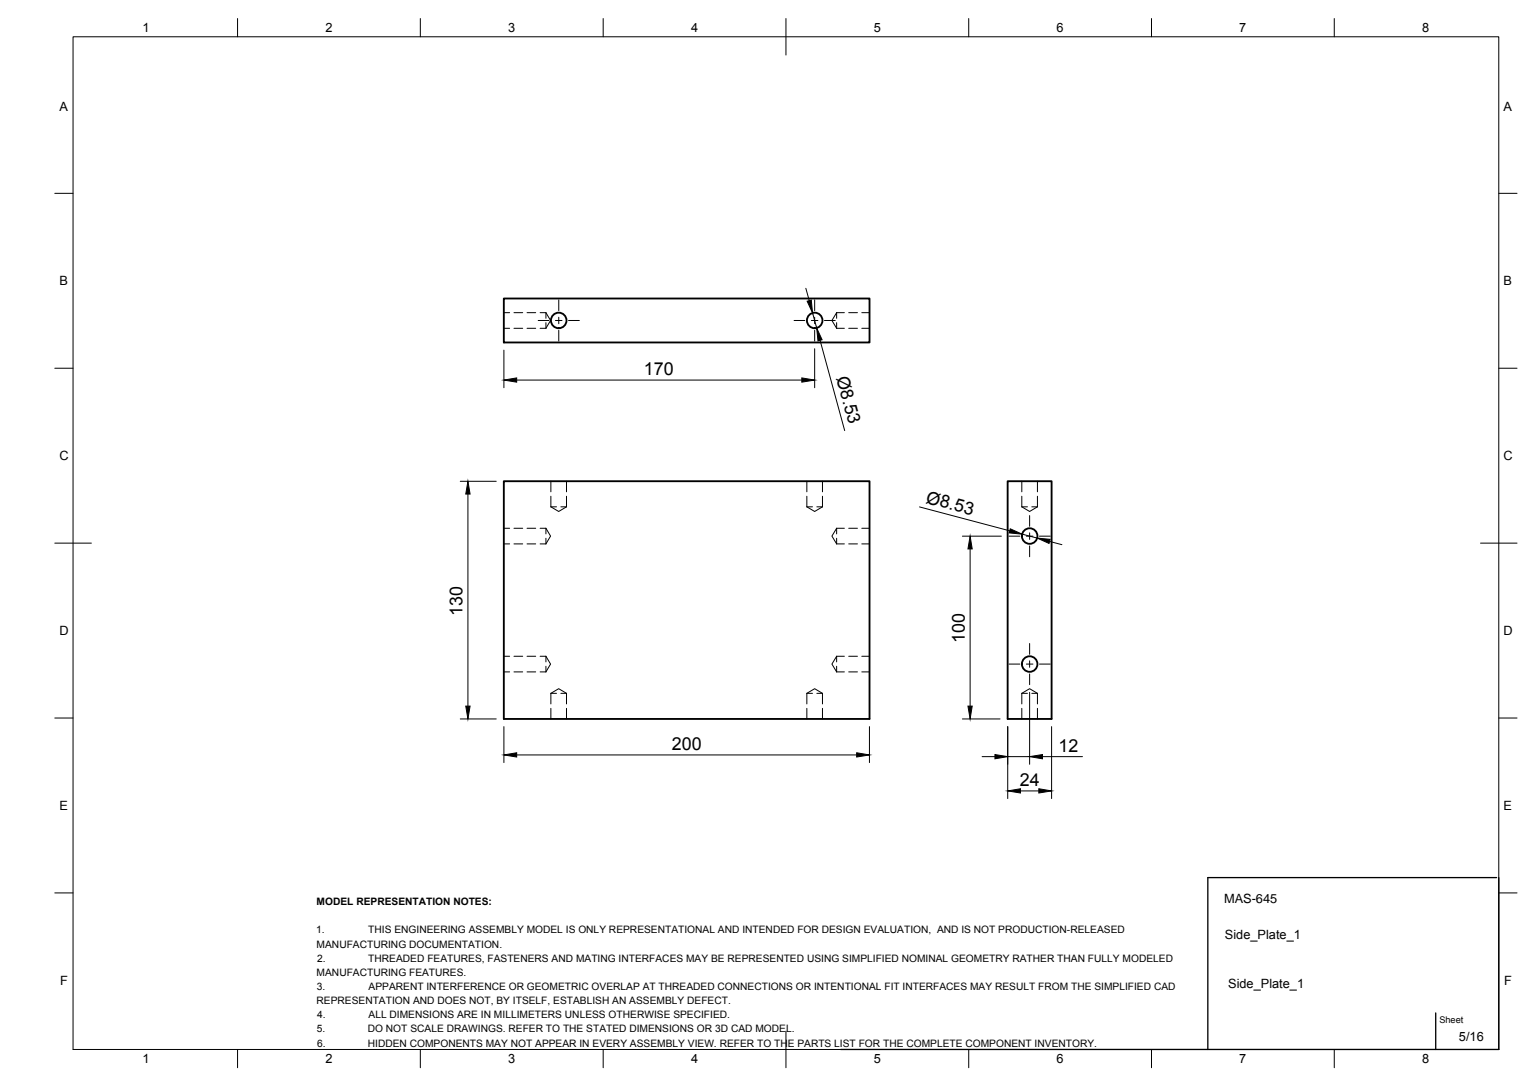
ISO-10303-21;
HEADER;
FILE_DESCRIPTION((''),'2;1');
FILE_NAME('Side_Plate_1.step','2026-10-09T10:54:55-07:00',(''),(''),'','','');
FILE_SCHEMA (('AUTOMOTIVE_DESIGN { 1 0 10303 214 3 1 1 }'));
ENDSEC;
DATA;
#10=MECHANICAL_DESIGN_GEOMETRIC_PRESENTATION_REPRESENTATION('',(#597),#63824);
#567=SHAPE_REPRESENTATION_RELATIONSHIP('SRR','None',#63881,#582) ;
#582=ADVANCED_BREP_SHAPE_REPRESENTATION('',(#612),#63811) ;
#597=STYLED_ITEM('',(#63963),#612) ;
#612=MANIFOLD_SOLID_BREP('Body1',#15496) ;
#687=FACE_BOUND('',#2566,.T.) ;
#688=FACE_BOUND('',#2567,.T.) ;
#689=FACE_BOUND('',#2574,.T.) ;
#690=FACE_BOUND('',#2575,.T.) ;
#691=FACE_BOUND('',#2578,.T.) ;
#692=FACE_BOUND('',#2579,.T.) ;
#693=FACE_BOUND('',#2581,.T.) ;
#694=FACE_BOUND('',#2582,.T.) ;
#860=PLANE('',#15878) ;
#861=PLANE('',#15887) ;
#862=PLANE('',#15888) ;
#863=PLANE('',#15889) ;
#864=PLANE('',#15890) ;
#865=PLANE('',#15891) ;
#1161=CYLINDRICAL_SURFACE('',#15856,4.263) ;
#1162=CYLINDRICAL_SURFACE('',#15860,4.263) ;
#1163=CYLINDRICAL_SURFACE('',#15864,4.263) ;
#1164=CYLINDRICAL_SURFACE('',#15868,4.263) ;
#1165=CYLINDRICAL_SURFACE('',#15872,4.263) ;
#1166=CYLINDRICAL_SURFACE('',#15876,4.263) ;
#1167=CYLINDRICAL_SURFACE('',#15881,4.263) ;
#1168=CYLINDRICAL_SURFACE('',#15885,4.263) ;
#1630=FACE_OUTER_BOUND('',#2553,.T.) ;
#1631=FACE_OUTER_BOUND('',#2554,.T.) ;
#1632=FACE_OUTER_BOUND('',#2555,.T.) ;
#1633=FACE_OUTER_BOUND('',#2556,.T.) ;
#1634=FACE_OUTER_BOUND('',#2557,.T.) ;
#1635=FACE_OUTER_BOUND('',#2558,.T.) ;
#1636=FACE_OUTER_BOUND('',#2559,.T.) ;
#1637=FACE_OUTER_BOUND('',#2560,.T.) ;
#1638=FACE_OUTER_BOUND('',#2561,.T.) ;
#1639=FACE_OUTER_BOUND('',#2562,.T.) ;
#1640=FACE_OUTER_BOUND('',#2563,.T.) ;
#1641=FACE_OUTER_BOUND('',#2564,.T.) ;
#1642=FACE_OUTER_BOUND('',#2565,.T.) ;
#1643=FACE_OUTER_BOUND('',#2568,.T.) ;
#1644=FACE_OUTER_BOUND('',#2569,.T.) ;
#1645=FACE_OUTER_BOUND('',#2570,.T.) ;
#1646=FACE_OUTER_BOUND('',#2571,.T.) ;
#1647=FACE_OUTER_BOUND('',#2572,.T.) ;
#1648=FACE_OUTER_BOUND('',#2573,.T.) ;
#1649=FACE_OUTER_BOUND('',#2576,.T.) ;
#1650=FACE_OUTER_BOUND('',#2577,.T.) ;
#1651=FACE_OUTER_BOUND('',#2580,.T.) ;
#2553=EDGE_LOOP('',(#10144,#10145,#10146)) ;
#2554=EDGE_LOOP('',(#10147,#10148,#10149,#10150)) ;
#2555=EDGE_LOOP('',(#10151,#10152,#10153)) ;
#2556=EDGE_LOOP('',(#10154,#10155,#10156,#10157)) ;
#2557=EDGE_LOOP('',(#10158,#10159,#10160)) ;
#2558=EDGE_LOOP('',(#10161,#10162,#10163,#10164)) ;
#2559=EDGE_LOOP('',(#10165,#10166,#10167)) ;
#2560=EDGE_LOOP('',(#10168,#10169,#10170,#10171)) ;
#2561=EDGE_LOOP('',(#10172,#10173,#10174)) ;
#2562=EDGE_LOOP('',(#10175,#10176,#10177,#10178)) ;
#2563=EDGE_LOOP('',(#10179,#10180,#10181)) ;
#2564=EDGE_LOOP('',(#10182,#10183,#10184,#10185)) ;
#2565=EDGE_LOOP('',(#10186,#10187,#10188,#10189)) ;
#2566=EDGE_LOOP('',(#10190)) ;
#2567=EDGE_LOOP('',(#10191)) ;
#2568=EDGE_LOOP('',(#10192,#10193,#10194)) ;
#2569=EDGE_LOOP('',(#10195,#10196,#10197,#10198)) ;
#2570=EDGE_LOOP('',(#10199,#10200,#10201)) ;
#2571=EDGE_LOOP('',(#10202,#10203,#10204,#10205)) ;
#2572=EDGE_LOOP('',(#10206,#10207,#10208,#10209)) ;
#2573=EDGE_LOOP('',(#10210,#10211,#10212,#10213)) ;
#2574=EDGE_LOOP('',(#10214)) ;
#2575=EDGE_LOOP('',(#10215)) ;
#2576=EDGE_LOOP('',(#10216,#10217,#10218,#10219)) ;
#2577=EDGE_LOOP('',(#10220,#10221,#10222,#10223)) ;
#2578=EDGE_LOOP('',(#10224)) ;
#2579=EDGE_LOOP('',(#10225)) ;
#2580=EDGE_LOOP('',(#10226,#10227,#10228,#10229)) ;
#2581=EDGE_LOOP('',(#10230)) ;
#2582=EDGE_LOOP('',(#10231)) ;
#3564=CIRCLE('',#15855,4.263) ;
#3565=CIRCLE('',#15857,4.263) ;
#3566=CIRCLE('',#15859,4.263) ;
#3567=CIRCLE('',#15861,4.263) ;
#3568=CIRCLE('',#15863,4.263) ;
#3569=CIRCLE('',#15865,4.263) ;
#3570=CIRCLE('',#15867,4.263) ;
#3571=CIRCLE('',#15869,4.263) ;
#3572=CIRCLE('',#15871,4.263) ;
#3573=CIRCLE('',#15873,4.263) ;
#3574=CIRCLE('',#15875,4.263) ;
#3575=CIRCLE('',#15877,4.263) ;
#3576=CIRCLE('',#15880,4.263) ;
#3577=CIRCLE('',#15882,4.263) ;
#3578=CIRCLE('',#15884,4.263) ;
#3579=CIRCLE('',#15886,4.263) ;
#4771=LINE('',#23393,#5427) ;
#4772=LINE('',#23398,#5428) ;
#4773=LINE('',#23402,#5429) ;
#4774=LINE('',#23407,#5430) ;
#4775=LINE('',#23411,#5431) ;
#4776=LINE('',#23416,#5432) ;
#4777=LINE('',#23420,#5433) ;
#4778=LINE('',#23425,#5434) ;
#4779=LINE('',#23429,#5435) ;
#4780=LINE('',#23433,#5436) ;
#4781=LINE('',#23438,#5437) ;
#4782=LINE('',#23442,#5438) ;
#4783=LINE('',#23447,#5439) ;
#4784=LINE('',#23449,#5440) ;
#4785=LINE('',#23451,#5441) ;
#4786=LINE('',#23452,#5442) ;
#4787=LINE('',#23456,#5443) ;
#4788=LINE('',#23461,#5444) ;
#4789=LINE('',#23465,#5445) ;
#4790=LINE('',#23470,#5446) ;
#4791=LINE('',#23474,#5447) ;
#4792=LINE('',#23475,#5448) ;
#4793=LINE('',#23476,#5449) ;
#4794=LINE('',#23479,#5450) ;
#4795=LINE('',#23480,#5451) ;
#4796=LINE('',#23483,#5452) ;
#4797=LINE('',#23484,#5453) ;
#4798=LINE('',#23486,#5454) ;
#5427=VECTOR('',#18343,2.42186816158307) ;
#5428=VECTOR('',#18350,4.263) ;
#5429=VECTOR('',#18353,2.42186816158307) ;
#5430=VECTOR('',#18360,4.263) ;
#5431=VECTOR('',#18363,2.42186816158307) ;
#5432=VECTOR('',#18370,4.263) ;
#5433=VECTOR('',#18373,2.42186816158307) ;
#5434=VECTOR('',#18380,4.263) ;
#5435=VECTOR('',#18383,2.42186816158307) ;
#5436=VECTOR('',#18388,4.263) ;
#5437=VECTOR('',#18393,2.42186816158307) ;
#5438=VECTOR('',#18398,4.263) ;
#5439=VECTOR('',#18403,10.) ;
#5440=VECTOR('',#18404,10.) ;
#5441=VECTOR('',#18405,10.) ;
#5442=VECTOR('',#18406,10.) ;
#5443=VECTOR('',#18409,2.42186816158307) ;
#5444=VECTOR('',#18416,4.263) ;
#5445=VECTOR('',#18419,2.42186816158307) ;
#5446=VECTOR('',#18426,4.263) ;
#5447=VECTOR('',#18429,10.) ;
#5448=VECTOR('',#18430,10.) ;
#5449=VECTOR('',#18431,10.) ;
#5450=VECTOR('',#18434,10.) ;
#5451=VECTOR('',#18435,10.) ;
#5452=VECTOR('',#18438,10.) ;
#5453=VECTOR('',#18439,10.) ;
#5454=VECTOR('',#18442,10.) ;
#6120=VERTEX_POINT('',#23391) ;
#6121=VERTEX_POINT('',#23392) ;
#6122=VERTEX_POINT('',#23396) ;
#6123=VERTEX_POINT('',#23400) ;
#6124=VERTEX_POINT('',#23401) ;
#6125=VERTEX_POINT('',#23405) ;
#6126=VERTEX_POINT('',#23409) ;
#6127=VERTEX_POINT('',#23410) ;
#6128=VERTEX_POINT('',#23414) ;
#6129=VERTEX_POINT('',#23418) ;
#6130=VERTEX_POINT('',#23419) ;
#6131=VERTEX_POINT('',#23423) ;
#6132=VERTEX_POINT('',#23427) ;
#6133=VERTEX_POINT('',#23428) ;
#6134=VERTEX_POINT('',#23432) ;
#6135=VERTEX_POINT('',#23436) ;
#6136=VERTEX_POINT('',#23437) ;
#6137=VERTEX_POINT('',#23441) ;
#6138=VERTEX_POINT('',#23445) ;
#6139=VERTEX_POINT('',#23446) ;
#6140=VERTEX_POINT('',#23448) ;
#6141=VERTEX_POINT('',#23450) ;
#6142=VERTEX_POINT('',#23454) ;
#6143=VERTEX_POINT('',#23455) ;
#6144=VERTEX_POINT('',#23459) ;
#6145=VERTEX_POINT('',#23463) ;
#6146=VERTEX_POINT('',#23464) ;
#6147=VERTEX_POINT('',#23468) ;
#6148=VERTEX_POINT('',#23472) ;
#6149=VERTEX_POINT('',#23473) ;
#6150=VERTEX_POINT('',#23478) ;
#6151=VERTEX_POINT('',#23482) ;
#7626=EDGE_CURVE('',#6120,#6121,#4771,.T.) ;
#7627=EDGE_CURVE('',#6121,#6121,#3564,.T.) ;
#7628=EDGE_CURVE('',#6122,#6122,#3565,.T.) ;
#7629=EDGE_CURVE('',#6122,#6121,#4772,.T.) ;
#7630=EDGE_CURVE('',#6123,#6124,#4773,.T.) ;
#7631=EDGE_CURVE('',#6124,#6124,#3566,.T.) ;
#7632=EDGE_CURVE('',#6125,#6125,#3567,.T.) ;
#7633=EDGE_CURVE('',#6125,#6124,#4774,.T.) ;
#7634=EDGE_CURVE('',#6126,#6127,#4775,.T.) ;
#7635=EDGE_CURVE('',#6127,#6127,#3568,.T.) ;
#7636=EDGE_CURVE('',#6128,#6128,#3569,.T.) ;
#7637=EDGE_CURVE('',#6128,#6127,#4776,.T.) ;
#7638=EDGE_CURVE('',#6129,#6130,#4777,.T.) ;
#7639=EDGE_CURVE('',#6130,#6130,#3570,.T.) ;
#7640=EDGE_CURVE('',#6131,#6131,#3571,.T.) ;
#7641=EDGE_CURVE('',#6131,#6130,#4778,.T.) ;
#7642=EDGE_CURVE('',#6132,#6133,#4779,.T.) ;
#7643=EDGE_CURVE('',#6133,#6133,#3572,.T.) ;
#7644=EDGE_CURVE('',#6133,#6134,#4780,.T.) ;
#7645=EDGE_CURVE('',#6134,#6134,#3573,.F.) ;
#7646=EDGE_CURVE('',#6135,#6136,#4781,.T.) ;
#7647=EDGE_CURVE('',#6136,#6136,#3574,.T.) ;
#7648=EDGE_CURVE('',#6136,#6137,#4782,.T.) ;
#7649=EDGE_CURVE('',#6137,#6137,#3575,.F.) ;
#7650=EDGE_CURVE('',#6138,#6139,#4783,.T.) ;
#7651=EDGE_CURVE('',#6140,#6138,#4784,.T.) ;
#7652=EDGE_CURVE('',#6141,#6140,#4785,.T.) ;
#7653=EDGE_CURVE('',#6139,#6141,#4786,.T.) ;
#7654=EDGE_CURVE('',#6142,#6143,#4787,.T.) ;
#7655=EDGE_CURVE('',#6143,#6143,#3576,.T.) ;
#7656=EDGE_CURVE('',#6144,#6144,#3577,.F.) ;
#7657=EDGE_CURVE('',#6144,#6143,#4788,.T.) ;
#7658=EDGE_CURVE('',#6145,#6146,#4789,.T.) ;
#7659=EDGE_CURVE('',#6146,#6146,#3578,.T.) ;
#7660=EDGE_CURVE('',#6147,#6147,#3579,.F.) ;
#7661=EDGE_CURVE('',#6147,#6146,#4790,.T.) ;
#7662=EDGE_CURVE('',#6148,#6149,#4791,.T.) ;
#7663=EDGE_CURVE('',#6148,#6139,#4792,.T.) ;
#7664=EDGE_CURVE('',#6149,#6141,#4793,.T.) ;
#7665=EDGE_CURVE('',#6149,#6150,#4794,.T.) ;
#7666=EDGE_CURVE('',#6150,#6140,#4795,.T.) ;
#7667=EDGE_CURVE('',#6150,#6151,#4796,.T.) ;
#7668=EDGE_CURVE('',#6151,#6138,#4797,.T.) ;
#7669=EDGE_CURVE('',#6151,#6148,#4798,.T.) ;
#10144=ORIENTED_EDGE('',*,*,#7626,.T.) ;
#10145=ORIENTED_EDGE('',*,*,#7627,.F.) ;
#10146=ORIENTED_EDGE('',*,*,#7626,.F.) ;
#10147=ORIENTED_EDGE('',*,*,#7628,.F.) ;
#10148=ORIENTED_EDGE('',*,*,#7629,.T.) ;
#10149=ORIENTED_EDGE('',*,*,#7627,.T.) ;
#10150=ORIENTED_EDGE('',*,*,#7629,.F.) ;
#10151=ORIENTED_EDGE('',*,*,#7630,.T.) ;
#10152=ORIENTED_EDGE('',*,*,#7631,.F.) ;
#10153=ORIENTED_EDGE('',*,*,#7630,.F.) ;
#10154=ORIENTED_EDGE('',*,*,#7632,.F.) ;
#10155=ORIENTED_EDGE('',*,*,#7633,.T.) ;
#10156=ORIENTED_EDGE('',*,*,#7631,.T.) ;
#10157=ORIENTED_EDGE('',*,*,#7633,.F.) ;
#10158=ORIENTED_EDGE('',*,*,#7634,.T.) ;
#10159=ORIENTED_EDGE('',*,*,#7635,.F.) ;
#10160=ORIENTED_EDGE('',*,*,#7634,.F.) ;
#10161=ORIENTED_EDGE('',*,*,#7636,.F.) ;
#10162=ORIENTED_EDGE('',*,*,#7637,.T.) ;
#10163=ORIENTED_EDGE('',*,*,#7635,.T.) ;
#10164=ORIENTED_EDGE('',*,*,#7637,.F.) ;
#10165=ORIENTED_EDGE('',*,*,#7638,.T.) ;
#10166=ORIENTED_EDGE('',*,*,#7639,.F.) ;
#10167=ORIENTED_EDGE('',*,*,#7638,.F.) ;
#10168=ORIENTED_EDGE('',*,*,#7640,.F.) ;
#10169=ORIENTED_EDGE('',*,*,#7641,.T.) ;
#10170=ORIENTED_EDGE('',*,*,#7639,.T.) ;
#10171=ORIENTED_EDGE('',*,*,#7641,.F.) ;
#10172=ORIENTED_EDGE('',*,*,#7642,.T.) ;
#10173=ORIENTED_EDGE('',*,*,#7643,.T.) ;
#10174=ORIENTED_EDGE('',*,*,#7642,.F.) ;
#10175=ORIENTED_EDGE('',*,*,#7643,.F.) ;
#10176=ORIENTED_EDGE('',*,*,#7644,.T.) ;
#10177=ORIENTED_EDGE('',*,*,#7645,.T.) ;
#10178=ORIENTED_EDGE('',*,*,#7644,.F.) ;
#10179=ORIENTED_EDGE('',*,*,#7646,.T.) ;
#10180=ORIENTED_EDGE('',*,*,#7647,.T.) ;
#10181=ORIENTED_EDGE('',*,*,#7646,.F.) ;
#10182=ORIENTED_EDGE('',*,*,#7647,.F.) ;
#10183=ORIENTED_EDGE('',*,*,#7648,.T.) ;
#10184=ORIENTED_EDGE('',*,*,#7649,.T.) ;
#10185=ORIENTED_EDGE('',*,*,#7648,.F.) ;
#10186=ORIENTED_EDGE('',*,*,#7650,.F.) ;
#10187=ORIENTED_EDGE('',*,*,#7651,.F.) ;
#10188=ORIENTED_EDGE('',*,*,#7652,.F.) ;
#10189=ORIENTED_EDGE('',*,*,#7653,.F.) ;
#10190=ORIENTED_EDGE('',*,*,#7645,.F.) ;
#10191=ORIENTED_EDGE('',*,*,#7649,.F.) ;
#10192=ORIENTED_EDGE('',*,*,#7654,.T.) ;
#10193=ORIENTED_EDGE('',*,*,#7655,.F.) ;
#10194=ORIENTED_EDGE('',*,*,#7654,.F.) ;
#10195=ORIENTED_EDGE('',*,*,#7656,.F.) ;
#10196=ORIENTED_EDGE('',*,*,#7657,.T.) ;
#10197=ORIENTED_EDGE('',*,*,#7655,.T.) ;
#10198=ORIENTED_EDGE('',*,*,#7657,.F.) ;
#10199=ORIENTED_EDGE('',*,*,#7658,.T.) ;
#10200=ORIENTED_EDGE('',*,*,#7659,.F.) ;
#10201=ORIENTED_EDGE('',*,*,#7658,.F.) ;
#10202=ORIENTED_EDGE('',*,*,#7660,.F.) ;
#10203=ORIENTED_EDGE('',*,*,#7661,.T.) ;
#10204=ORIENTED_EDGE('',*,*,#7659,.T.) ;
#10205=ORIENTED_EDGE('',*,*,#7661,.F.) ;
#10206=ORIENTED_EDGE('',*,*,#7662,.F.) ;
#10207=ORIENTED_EDGE('',*,*,#7663,.T.) ;
#10208=ORIENTED_EDGE('',*,*,#7653,.T.) ;
#10209=ORIENTED_EDGE('',*,*,#7664,.F.) ;
#10210=ORIENTED_EDGE('',*,*,#7665,.F.) ;
#10211=ORIENTED_EDGE('',*,*,#7664,.T.) ;
#10212=ORIENTED_EDGE('',*,*,#7652,.T.) ;
#10213=ORIENTED_EDGE('',*,*,#7666,.F.) ;
#10214=ORIENTED_EDGE('',*,*,#7628,.T.) ;
#10215=ORIENTED_EDGE('',*,*,#7632,.T.) ;
#10216=ORIENTED_EDGE('',*,*,#7667,.F.) ;
#10217=ORIENTED_EDGE('',*,*,#7666,.T.) ;
#10218=ORIENTED_EDGE('',*,*,#7651,.T.) ;
#10219=ORIENTED_EDGE('',*,*,#7668,.F.) ;
#10220=ORIENTED_EDGE('',*,*,#7669,.F.) ;
#10221=ORIENTED_EDGE('',*,*,#7668,.T.) ;
#10222=ORIENTED_EDGE('',*,*,#7650,.T.) ;
#10223=ORIENTED_EDGE('',*,*,#7663,.F.) ;
#10224=ORIENTED_EDGE('',*,*,#7636,.T.) ;
#10225=ORIENTED_EDGE('',*,*,#7640,.T.) ;
#10226=ORIENTED_EDGE('',*,*,#7669,.T.) ;
#10227=ORIENTED_EDGE('',*,*,#7662,.T.) ;
#10228=ORIENTED_EDGE('',*,*,#7665,.T.) ;
#10229=ORIENTED_EDGE('',*,*,#7667,.T.) ;
#10230=ORIENTED_EDGE('',*,*,#7656,.T.) ;
#10231=ORIENTED_EDGE('',*,*,#7660,.T.) ;
#14508=CONICAL_SURFACE('',#15854,2.42186816158307,1.02974425867665) ;
#14509=CONICAL_SURFACE('',#15858,2.42186816158307,1.02974425867665) ;
#14510=CONICAL_SURFACE('',#15862,2.42186816158307,1.02974425867665) ;
#14511=CONICAL_SURFACE('',#15866,2.42186816158307,1.02974425867665) ;
#14512=CONICAL_SURFACE('',#15870,2.42186816158307,1.02974425867665) ;
#14513=CONICAL_SURFACE('',#15874,2.42186816158307,1.02974425867665) ;
#14514=CONICAL_SURFACE('',#15879,2.42186816158307,1.02974425867665) ;
#14515=CONICAL_SURFACE('',#15883,2.42186816158307,1.02974425867665) ;
#14718=ADVANCED_FACE('',(#1630),#14508,.F.) ;
#14719=ADVANCED_FACE('',(#1631),#1161,.F.) ;
#14720=ADVANCED_FACE('',(#1632),#14509,.F.) ;
#14721=ADVANCED_FACE('',(#1633),#1162,.F.) ;
#14722=ADVANCED_FACE('',(#1634),#14510,.F.) ;
#14723=ADVANCED_FACE('',(#1635),#1163,.F.) ;
#14724=ADVANCED_FACE('',(#1636),#14511,.F.) ;
#14725=ADVANCED_FACE('',(#1637),#1164,.F.) ;
#14726=ADVANCED_FACE('',(#1638),#14512,.F.) ;
#14727=ADVANCED_FACE('',(#1639),#1165,.F.) ;
#14728=ADVANCED_FACE('',(#1640),#14513,.F.) ;
#14729=ADVANCED_FACE('',(#1641),#1166,.F.) ;
#14730=ADVANCED_FACE('',(#1642,#687,#688),#860,.T.) ;
#14731=ADVANCED_FACE('',(#1643),#14514,.F.) ;
#14732=ADVANCED_FACE('',(#1644),#1167,.F.) ;
#14733=ADVANCED_FACE('',(#1645),#14515,.F.) ;
#14734=ADVANCED_FACE('',(#1646),#1168,.F.) ;
#14735=ADVANCED_FACE('',(#1647),#861,.T.) ;
#14736=ADVANCED_FACE('',(#1648,#689,#690),#862,.T.) ;
#14737=ADVANCED_FACE('',(#1649),#863,.T.) ;
#14738=ADVANCED_FACE('',(#1650,#691,#692),#864,.T.) ;
#14739=ADVANCED_FACE('',(#1651,#693,#694),#865,.F.) ;
#15496=CLOSED_SHELL('',(#14718,#14719,#14720,#14721,#14722,#14723,#14724,
#14725,#14726,#14727,#14728,#14729,#14730,#14731,#14732,#14733,#14734,#14735,
#14736,#14737,#14738,#14739)) ;
#15853=AXIS2_PLACEMENT_3D('',#23389,#18339,#18340) ;
#15854=AXIS2_PLACEMENT_3D('',#23390,#18341,#18342) ;
#15855=AXIS2_PLACEMENT_3D('',#23394,#18344,#18345) ;
#15856=AXIS2_PLACEMENT_3D('',#23395,#18346,#18347) ;
#15857=AXIS2_PLACEMENT_3D('',#23397,#18348,#18349) ;
#15858=AXIS2_PLACEMENT_3D('',#23399,#18351,#18352) ;
#15859=AXIS2_PLACEMENT_3D('',#23403,#18354,#18355) ;
#15860=AXIS2_PLACEMENT_3D('',#23404,#18356,#18357) ;
#15861=AXIS2_PLACEMENT_3D('',#23406,#18358,#18359) ;
#15862=AXIS2_PLACEMENT_3D('',#23408,#18361,#18362) ;
#15863=AXIS2_PLACEMENT_3D('',#23412,#18364,#18365) ;
#15864=AXIS2_PLACEMENT_3D('',#23413,#18366,#18367) ;
#15865=AXIS2_PLACEMENT_3D('',#23415,#18368,#18369) ;
#15866=AXIS2_PLACEMENT_3D('',#23417,#18371,#18372) ;
#15867=AXIS2_PLACEMENT_3D('',#23421,#18374,#18375) ;
#15868=AXIS2_PLACEMENT_3D('',#23422,#18376,#18377) ;
#15869=AXIS2_PLACEMENT_3D('',#23424,#18378,#18379) ;
#15870=AXIS2_PLACEMENT_3D('',#23426,#18381,#18382) ;
#15871=AXIS2_PLACEMENT_3D('',#23430,#18384,#18385) ;
#15872=AXIS2_PLACEMENT_3D('',#23431,#18386,#18387) ;
#15873=AXIS2_PLACEMENT_3D('',#23434,#18389,#18390) ;
#15874=AXIS2_PLACEMENT_3D('',#23435,#18391,#18392) ;
#15875=AXIS2_PLACEMENT_3D('',#23439,#18394,#18395) ;
#15876=AXIS2_PLACEMENT_3D('',#23440,#18396,#18397) ;
#15877=AXIS2_PLACEMENT_3D('',#23443,#18399,#18400) ;
#15878=AXIS2_PLACEMENT_3D('',#23444,#18401,#18402) ;
#15879=AXIS2_PLACEMENT_3D('',#23453,#18407,#18408) ;
#15880=AXIS2_PLACEMENT_3D('',#23457,#18410,#18411) ;
#15881=AXIS2_PLACEMENT_3D('',#23458,#18412,#18413) ;
#15882=AXIS2_PLACEMENT_3D('',#23460,#18414,#18415) ;
#15883=AXIS2_PLACEMENT_3D('',#23462,#18417,#18418) ;
#15884=AXIS2_PLACEMENT_3D('',#23466,#18420,#18421) ;
#15885=AXIS2_PLACEMENT_3D('',#23467,#18422,#18423) ;
#15886=AXIS2_PLACEMENT_3D('',#23469,#18424,#18425) ;
#15887=AXIS2_PLACEMENT_3D('',#23471,#18427,#18428) ;
#15888=AXIS2_PLACEMENT_3D('',#23477,#18432,#18433) ;
#15889=AXIS2_PLACEMENT_3D('',#23481,#18436,#18437) ;
#15890=AXIS2_PLACEMENT_3D('',#23485,#18440,#18441) ;
#15891=AXIS2_PLACEMENT_3D('',#23487,#18443,#18444) ;
#18339=DIRECTION('axis',(0.,0.,1.)) ;
#18340=DIRECTION('refdir',(1.,0.,0.)) ;
#18341=DIRECTION('center_axis',(-9.473903143468E-16,1.,0.)) ;
#18342=DIRECTION('ref_axis',(0.,0.,1.)) ;
#18343=DIRECTION('',(-5.92914802803472E-16,0.515038074910058,-0.85716730070211)) ;
#18344=DIRECTION('center_axis',(9.473903143468E-16,-1.,0.)) ;
#18345=DIRECTION('ref_axis',(0.,0.,1.)) ;
#18346=DIRECTION('center_axis',(9.473903143468E-16,-1.,0.)) ;
#18347=DIRECTION('ref_axis',(0.,0.,1.)) ;
#18348=DIRECTION('center_axis',(9.47390314346801E-16,-1.,0.)) ;
#18349=DIRECTION('ref_axis',(0.,0.,1.)) ;
#18350=DIRECTION('',(9.473903143468E-16,-1.,0.)) ;
#18351=DIRECTION('center_axis',(-9.473903143468E-16,1.,0.)) ;
#18352=DIRECTION('ref_axis',(0.,0.,1.)) ;
#18353=DIRECTION('',(-5.92914802803472E-16,0.515038074910058,-0.85716730070211)) ;
#18354=DIRECTION('center_axis',(9.473903143468E-16,-1.,0.)) ;
#18355=DIRECTION('ref_axis',(0.,0.,1.)) ;
#18356=DIRECTION('center_axis',(9.473903143468E-16,-1.,0.)) ;
#18357=DIRECTION('ref_axis',(0.,0.,1.)) ;
#18358=DIRECTION('center_axis',(9.47390314346801E-16,-1.,0.)) ;
#18359=DIRECTION('ref_axis',(0.,0.,1.)) ;
#18360=DIRECTION('',(9.473903143468E-16,-1.,0.)) ;
#18361=DIRECTION('center_axis',(-3.5527136788005E-16,-1.,0.)) ;
#18362=DIRECTION('ref_axis',(0.,0.,-1.)) ;
#18363=DIRECTION('',(-2.87951000497466E-16,-0.515038074910058,0.85716730070211)) ;
#18364=DIRECTION('center_axis',(3.5527136788005E-16,1.,0.)) ;
#18365=DIRECTION('ref_axis',(0.,0.,-1.)) ;
#18366=DIRECTION('center_axis',(3.5527136788005E-16,1.,0.)) ;
#18367=DIRECTION('ref_axis',(0.,0.,-1.)) ;
#18368=DIRECTION('center_axis',(4.2632564145606E-15,1.,0.)) ;
#18369=DIRECTION('ref_axis',(0.,0.,-1.)) ;
#18370=DIRECTION('',(3.5527136788005E-16,1.,0.)) ;
#18371=DIRECTION('center_axis',(-3.5527136788005E-16,-1.,0.)) ;
#18372=DIRECTION('ref_axis',(0.,0.,-1.)) ;
#18373=DIRECTION('',(-2.87951000497466E-16,-0.515038074910058,0.85716730070211)) ;
#18374=DIRECTION('center_axis',(3.5527136788005E-16,1.,0.)) ;
#18375=DIRECTION('ref_axis',(0.,0.,-1.)) ;
#18376=DIRECTION('center_axis',(3.5527136788005E-16,1.,0.)) ;
#18377=DIRECTION('ref_axis',(0.,0.,-1.)) ;
#18378=DIRECTION('center_axis',(4.2632564145606E-15,1.,0.)) ;
#18379=DIRECTION('ref_axis',(0.,0.,-1.)) ;
#18380=DIRECTION('',(3.5527136788005E-16,1.,0.)) ;
#18381=DIRECTION('center_axis',(0.,0.,-1.)) ;
#18382=DIRECTION('ref_axis',(1.,0.,0.)) ;
#18383=DIRECTION('',(-0.85716730070211,1.04972719113862E-16,-0.515038074910058)) ;
#18384=DIRECTION('center_axis',(0.,0.,-1.)) ;
#18385=DIRECTION('ref_axis',(1.,0.,0.)) ;
#18386=DIRECTION('center_axis',(0.,0.,-1.)) ;
#18387=DIRECTION('ref_axis',(1.,0.,0.)) ;
#18388=DIRECTION('',(0.,0.,-1.)) ;
#18389=DIRECTION('center_axis',(0.,0.,1.)) ;
#18390=DIRECTION('ref_axis',(1.,0.,0.)) ;
#18391=DIRECTION('center_axis',(0.,0.,-1.)) ;
#18392=DIRECTION('ref_axis',(1.,0.,0.)) ;
#18393=DIRECTION('',(-0.85716730070211,1.04972719113862E-16,-0.515038074910058)) ;
#18394=DIRECTION('center_axis',(0.,0.,-1.)) ;
#18395=DIRECTION('ref_axis',(1.,0.,0.)) ;
#18396=DIRECTION('center_axis',(0.,0.,-1.)) ;
#18397=DIRECTION('ref_axis',(1.,0.,0.)) ;
#18398=DIRECTION('',(0.,0.,-1.)) ;
#18399=DIRECTION('center_axis',(0.,0.,1.)) ;
#18400=DIRECTION('ref_axis',(1.,0.,0.)) ;
#18401=DIRECTION('center_axis',(0.,0.,-1.)) ;
#18402=DIRECTION('ref_axis',(-1.,0.,0.)) ;
#18403=DIRECTION('',(1.,-4.2632564145606E-15,0.)) ;
#18404=DIRECTION('',(1.02140518265514E-15,-1.,0.)) ;
#18405=DIRECTION('',(-1.,-9.47390314346801E-16,0.)) ;
#18406=DIRECTION('',(2.66453525910036E-16,1.,0.)) ;
#18407=DIRECTION('center_axis',(0.,0.,1.)) ;
#18408=DIRECTION('ref_axis',(1.,0.,0.)) ;
#18409=DIRECTION('',(-0.85716730070211,-1.04972719113862E-16,0.515038074910058)) ;
#18410=DIRECTION('center_axis',(0.,0.,-1.)) ;
#18411=DIRECTION('ref_axis',(1.,0.,0.)) ;
#18412=DIRECTION('center_axis',(0.,0.,-1.)) ;
#18413=DIRECTION('ref_axis',(1.,0.,0.)) ;
#18414=DIRECTION('center_axis',(0.,0.,1.)) ;
#18415=DIRECTION('ref_axis',(1.,0.,0.)) ;
#18416=DIRECTION('',(0.,0.,-1.)) ;
#18417=DIRECTION('center_axis',(0.,0.,1.)) ;
#18418=DIRECTION('ref_axis',(1.,0.,0.)) ;
#18419=DIRECTION('',(-0.85716730070211,-1.04972719113862E-16,0.515038074910058)) ;
#18420=DIRECTION('center_axis',(0.,0.,-1.)) ;
#18421=DIRECTION('ref_axis',(1.,0.,0.)) ;
#18422=DIRECTION('center_axis',(0.,0.,-1.)) ;
#18423=DIRECTION('ref_axis',(1.,0.,0.)) ;
#18424=DIRECTION('center_axis',(0.,0.,1.)) ;
#18425=DIRECTION('ref_axis',(1.,0.,0.)) ;
#18426=DIRECTION('',(0.,0.,-1.)) ;
#18427=DIRECTION('center_axis',(1.,-2.66453525910036E-16,0.)) ;
#18428=DIRECTION('ref_axis',(-2.66453525910036E-16,-1.,0.)) ;
#18429=DIRECTION('',(2.66453525910036E-16,1.,0.)) ;
#18430=DIRECTION('',(0.,0.,-1.)) ;
#18431=DIRECTION('',(0.,0.,-1.)) ;
#18432=DIRECTION('center_axis',(-9.47390314346801E-16,1.,0.)) ;
#18433=DIRECTION('ref_axis',(1.,9.47390314346801E-16,0.)) ;
#18434=DIRECTION('',(-1.,-9.47390314346801E-16,0.)) ;
#18435=DIRECTION('',(0.,0.,-1.)) ;
#18436=DIRECTION('center_axis',(-1.,-1.02140518265514E-15,0.)) ;
#18437=DIRECTION('ref_axis',(-1.02140518265514E-15,1.,0.)) ;
#18438=DIRECTION('',(1.02140518265514E-15,-1.,0.)) ;
#18439=DIRECTION('',(0.,0.,-1.)) ;
#18440=DIRECTION('center_axis',(-4.2632564145606E-15,-1.,0.)) ;
#18441=DIRECTION('ref_axis',(-1.,4.2632564145606E-15,0.)) ;
#18442=DIRECTION('',(1.,-4.2632564145606E-15,0.)) ;
#18443=DIRECTION('center_axis',(0.,0.,-1.)) ;
#18444=DIRECTION('ref_axis',(-1.,0.,0.)) ;
#23389=CARTESIAN_POINT('',(0.,0.,0.)) ;
#23390=CARTESIAN_POINT('Origin',(62.9999999999988,385.343736383858,-54.)) ;
#23391=CARTESIAN_POINT('',(62.9999999999988,383.888531181086,-54.)) ;
#23392=CARTESIAN_POINT('',(62.9999999999988,386.45,-58.263)) ;
#23393=CARTESIAN_POINT('',(62.9999999999988,385.343736383858,-56.4218681615831)) ;
#23394=CARTESIAN_POINT('Origin',(62.9999999999988,386.45,-54.)) ;
#23395=CARTESIAN_POINT('Origin',(62.9999999999988,405.45,-54.)) ;
#23396=CARTESIAN_POINT('',(62.9999999999988,409.45,-58.263)) ;
#23397=CARTESIAN_POINT('Origin',(62.9999999999988,409.45,-54.)) ;
#23398=CARTESIAN_POINT('',(62.9999999999988,405.45,-58.263)) ;
#23399=CARTESIAN_POINT('Origin',(62.9999999999988,385.343736383858,-124.)) ;
#23400=CARTESIAN_POINT('',(62.9999999999988,383.888531181086,-124.)) ;
#23401=CARTESIAN_POINT('',(62.9999999999988,386.45,-128.263)) ;
#23402=CARTESIAN_POINT('',(62.9999999999988,385.343736383858,-126.421868161583)) ;
#23403=CARTESIAN_POINT('Origin',(62.9999999999988,386.45,-124.)) ;
#23404=CARTESIAN_POINT('Origin',(62.9999999999988,405.45,-124.)) ;
#23405=CARTESIAN_POINT('',(62.9999999999988,409.45,-128.263)) ;
#23406=CARTESIAN_POINT('Origin',(62.9999999999988,409.45,-124.)) ;
#23407=CARTESIAN_POINT('',(62.9999999999988,405.45,-128.263)) ;
#23408=CARTESIAN_POINT('Origin',(62.9999999999994,228.556263616143,-124.)) ;
#23409=CARTESIAN_POINT('',(62.9999999999994,230.011468818914,-124.)) ;
#23410=CARTESIAN_POINT('',(62.9999999999994,227.45,-119.737)) ;
#23411=CARTESIAN_POINT('',(62.9999999999994,228.556263616143,-121.578131838417)) ;
#23412=CARTESIAN_POINT('Origin',(62.9999999999994,227.45,-124.)) ;
#23413=CARTESIAN_POINT('Origin',(62.9999999999994,208.45,-124.)) ;
#23414=CARTESIAN_POINT('',(62.9999999999994,209.449999999999,-119.737)) ;
#23415=CARTESIAN_POINT('Origin',(62.9999999999994,209.449999999999,-124.)) ;
#23416=CARTESIAN_POINT('',(62.9999999999994,208.45,-119.737)) ;
#23417=CARTESIAN_POINT('Origin',(62.9999999999994,228.556263616143,-54.)) ;
#23418=CARTESIAN_POINT('',(62.9999999999994,230.011468818914,-54.)) ;
#23419=CARTESIAN_POINT('',(62.9999999999994,227.45,-49.737)) ;
#23420=CARTESIAN_POINT('',(62.9999999999994,228.556263616143,-51.5781318384169)) ;
#23421=CARTESIAN_POINT('Origin',(62.9999999999994,227.45,-54.)) ;
#23422=CARTESIAN_POINT('Origin',(62.9999999999994,208.45,-54.)) ;
#23423=CARTESIAN_POINT('',(62.9999999999994,209.449999999999,-49.737)) ;
#23424=CARTESIAN_POINT('Origin',(62.9999999999994,209.449999999999,-54.)) ;
#23425=CARTESIAN_POINT('',(62.9999999999994,208.45,-49.737)) ;
#23426=CARTESIAN_POINT('Origin',(63.,379.45,-138.893736383857)) ;
#23427=CARTESIAN_POINT('',(63.,379.45,-137.438531181086)) ;
#23428=CARTESIAN_POINT('',(58.737,379.45,-140.)) ;
#23429=CARTESIAN_POINT('',(60.5781318384169,379.45,-138.893736383857)) ;
#23430=CARTESIAN_POINT('Origin',(63.,379.45,-140.)) ;
#23431=CARTESIAN_POINT('Origin',(63.,379.45,-159.)) ;
#23432=CARTESIAN_POINT('',(58.737,379.45,-154.)) ;
#23433=CARTESIAN_POINT('',(58.737,379.45,-159.)) ;
#23434=CARTESIAN_POINT('Origin',(63.,379.45,-154.)) ;
#23435=CARTESIAN_POINT('Origin',(63.,239.45,-138.893736383857)) ;
#23436=CARTESIAN_POINT('',(63.,239.45,-137.438531181086)) ;
#23437=CARTESIAN_POINT('',(58.737,239.45,-140.)) ;
#23438=CARTESIAN_POINT('',(60.5781318384169,239.45,-138.893736383857)) ;
#23439=CARTESIAN_POINT('Origin',(63.,239.45,-140.)) ;
#23440=CARTESIAN_POINT('Origin',(63.,239.45,-159.)) ;
#23441=CARTESIAN_POINT('',(58.737,239.45,-154.)) ;
#23442=CARTESIAN_POINT('',(58.737,239.45,-159.)) ;
#23443=CARTESIAN_POINT('Origin',(63.,239.45,-154.)) ;
#23444=CARTESIAN_POINT('Origin',(63.,309.45,-154.)) ;
#23445=CARTESIAN_POINT('',(51.0000000000001,209.449999999999,-154.)) ;
#23446=CARTESIAN_POINT('',(75.,209.449999999999,-154.)) ;
#23447=CARTESIAN_POINT('',(68.9999999999998,209.449999999999,-154.)) ;
#23448=CARTESIAN_POINT('',(50.9999999999999,409.45,-154.)) ;
#23449=CARTESIAN_POINT('',(51.0000000000001,259.449999999999,-154.)) ;
#23450=CARTESIAN_POINT('',(75.0000000000001,409.45,-154.)) ;
#23451=CARTESIAN_POINT('',(56.9999999999999,409.45,-154.)) ;
#23452=CARTESIAN_POINT('',(75.0000000000001,359.45,-154.)) ;
#23453=CARTESIAN_POINT('Origin',(63.,379.45,-39.1062636161425)) ;
#23454=CARTESIAN_POINT('',(63.,379.45,-40.5614688189145)) ;
#23455=CARTESIAN_POINT('',(58.737,379.45,-38.)) ;
#23456=CARTESIAN_POINT('',(60.5781318384169,379.45,-39.1062636161425)) ;
#23457=CARTESIAN_POINT('Origin',(63.,379.45,-38.)) ;
#23458=CARTESIAN_POINT('Origin',(63.,379.45,-19.)) ;
#23459=CARTESIAN_POINT('',(58.737,379.45,-24.)) ;
#23460=CARTESIAN_POINT('Origin',(63.,379.45,-24.)) ;
#23461=CARTESIAN_POINT('',(58.737,379.45,-19.)) ;
#23462=CARTESIAN_POINT('Origin',(63.,239.45,-39.1062636161425)) ;
#23463=CARTESIAN_POINT('',(63.,239.45,-40.5614688189145)) ;
#23464=CARTESIAN_POINT('',(58.737,239.45,-38.)) ;
#23465=CARTESIAN_POINT('',(60.5781318384169,239.45,-39.1062636161425)) ;
#23466=CARTESIAN_POINT('Origin',(63.,239.45,-38.)) ;
#23467=CARTESIAN_POINT('Origin',(63.,239.45,-19.)) ;
#23468=CARTESIAN_POINT('',(58.737,239.45,-24.)) ;
#23469=CARTESIAN_POINT('Origin',(63.,239.45,-24.)) ;
#23470=CARTESIAN_POINT('',(58.737,239.45,-19.)) ;
#23471=CARTESIAN_POINT('Origin',(75.0000000000001,409.45,-24.)) ;
#23472=CARTESIAN_POINT('',(75.,209.449999999999,-24.)) ;
#23473=CARTESIAN_POINT('',(75.0000000000001,409.45,-24.)) ;
#23474=CARTESIAN_POINT('',(75.0000000000001,359.45,-24.)) ;
#23475=CARTESIAN_POINT('',(75.,209.449999999999,-24.)) ;
#23476=CARTESIAN_POINT('',(75.0000000000001,409.45,-24.)) ;
#23477=CARTESIAN_POINT('Origin',(50.9999999999999,409.45,-24.)) ;
#23478=CARTESIAN_POINT('',(50.9999999999999,409.45,-24.)) ;
#23479=CARTESIAN_POINT('',(56.9999999999999,409.45,-24.)) ;
#23480=CARTESIAN_POINT('',(50.9999999999999,409.45,-24.)) ;
#23481=CARTESIAN_POINT('Origin',(51.0000000000001,209.449999999999,-24.)) ;
#23482=CARTESIAN_POINT('',(51.0000000000001,209.449999999999,-24.)) ;
#23483=CARTESIAN_POINT('',(51.0000000000001,259.449999999999,-24.)) ;
#23484=CARTESIAN_POINT('',(51.0000000000001,209.449999999999,-24.)) ;
#23485=CARTESIAN_POINT('Origin',(75.,209.449999999999,-24.)) ;
#23486=CARTESIAN_POINT('',(68.9999999999998,209.449999999999,-24.)) ;
#23487=CARTESIAN_POINT('Origin',(63.,309.45,-24.)) ;
#63794=UNCERTAINTY_MEASURE_WITH_UNIT(LENGTH_MEASURE(0.01),#63825,
'DISTANCE_ACCURACY_VALUE',
'Maximum model space distance between geometric entities at asserted c
onnectivities') ;
#63807=UNCERTAINTY_MEASURE_WITH_UNIT(LENGTH_MEASURE(0.01),#63825,
'DISTANCE_ACCURACY_VALUE',
'Maximum model space distance between geometric entities at asserted c
onnectivities') ;
#63811=(
GEOMETRIC_REPRESENTATION_CONTEXT(3)
GLOBAL_UNCERTAINTY_ASSIGNED_CONTEXT((#63794))
GLOBAL_UNIT_ASSIGNED_CONTEXT((#63825,#63827,#63828))
REPRESENTATION_CONTEXT('','3D')
) ;
#63824=(
GEOMETRIC_REPRESENTATION_CONTEXT(3)
GLOBAL_UNCERTAINTY_ASSIGNED_CONTEXT((#63807))
GLOBAL_UNIT_ASSIGNED_CONTEXT((#63825,#63827,#63828))
REPRESENTATION_CONTEXT('','3D')
) ;
#63825=(
LENGTH_UNIT()
NAMED_UNIT(*)
SI_UNIT(.MILLI.,.METRE.)
) ;
#63827=(
NAMED_UNIT(*)
PLANE_ANGLE_UNIT()
SI_UNIT($,.RADIAN.)
) ;
#63828=(
NAMED_UNIT(*)
SI_UNIT($,.STERADIAN.)
SOLID_ANGLE_UNIT()
) ;
#63832=SHAPE_DEFINITION_REPRESENTATION(#63848,#63881) ;
#63848=PRODUCT_DEFINITION_SHAPE('',$,#63898) ;
#63881=SHAPE_REPRESENTATION('',(#15853),#63811) ;
#63894=PRODUCT_DEFINITION_CONTEXT('part definition',#63944,'design') ;
#63898=PRODUCT_DEFINITION('Side_Plate_1','Side_Plate_1',#63914,#63894) ;
#63914=PRODUCT_DEFINITION_FORMATION('',$,#63949) ;
#63944=APPLICATION_CONTEXT(
'Core Data for Automotive Mechanical Design Process') ;
#63945=PRODUCT_CONTEXT('part definition',#63944,'mechanical') ;
#63949=PRODUCT('Side_Plate_1','Side_Plate_1',$,(#63945)) ;
#63963=PRESENTATION_STYLE_ASSIGNMENT((#63968)) ;
#63968=SURFACE_STYLE_USAGE(.BOTH.,#63973) ;
#63973=SURFACE_SIDE_STYLE('',(#63978)) ;
#63978=SURFACE_STYLE_FILL_AREA(#63983) ;
#63983=FILL_AREA_STYLE('Opaque(160,160,160)',(#63988)) ;
#63988=FILL_AREA_STYLE_COLOUR('Opaque(160,160,160)',#63993) ;
#63993=COLOUR_RGB('Opaque(160,160,160)', 0.09019608, 0.27058824, 0.51372549) ;
ENDSEC;
END-ISO-10303-21;
